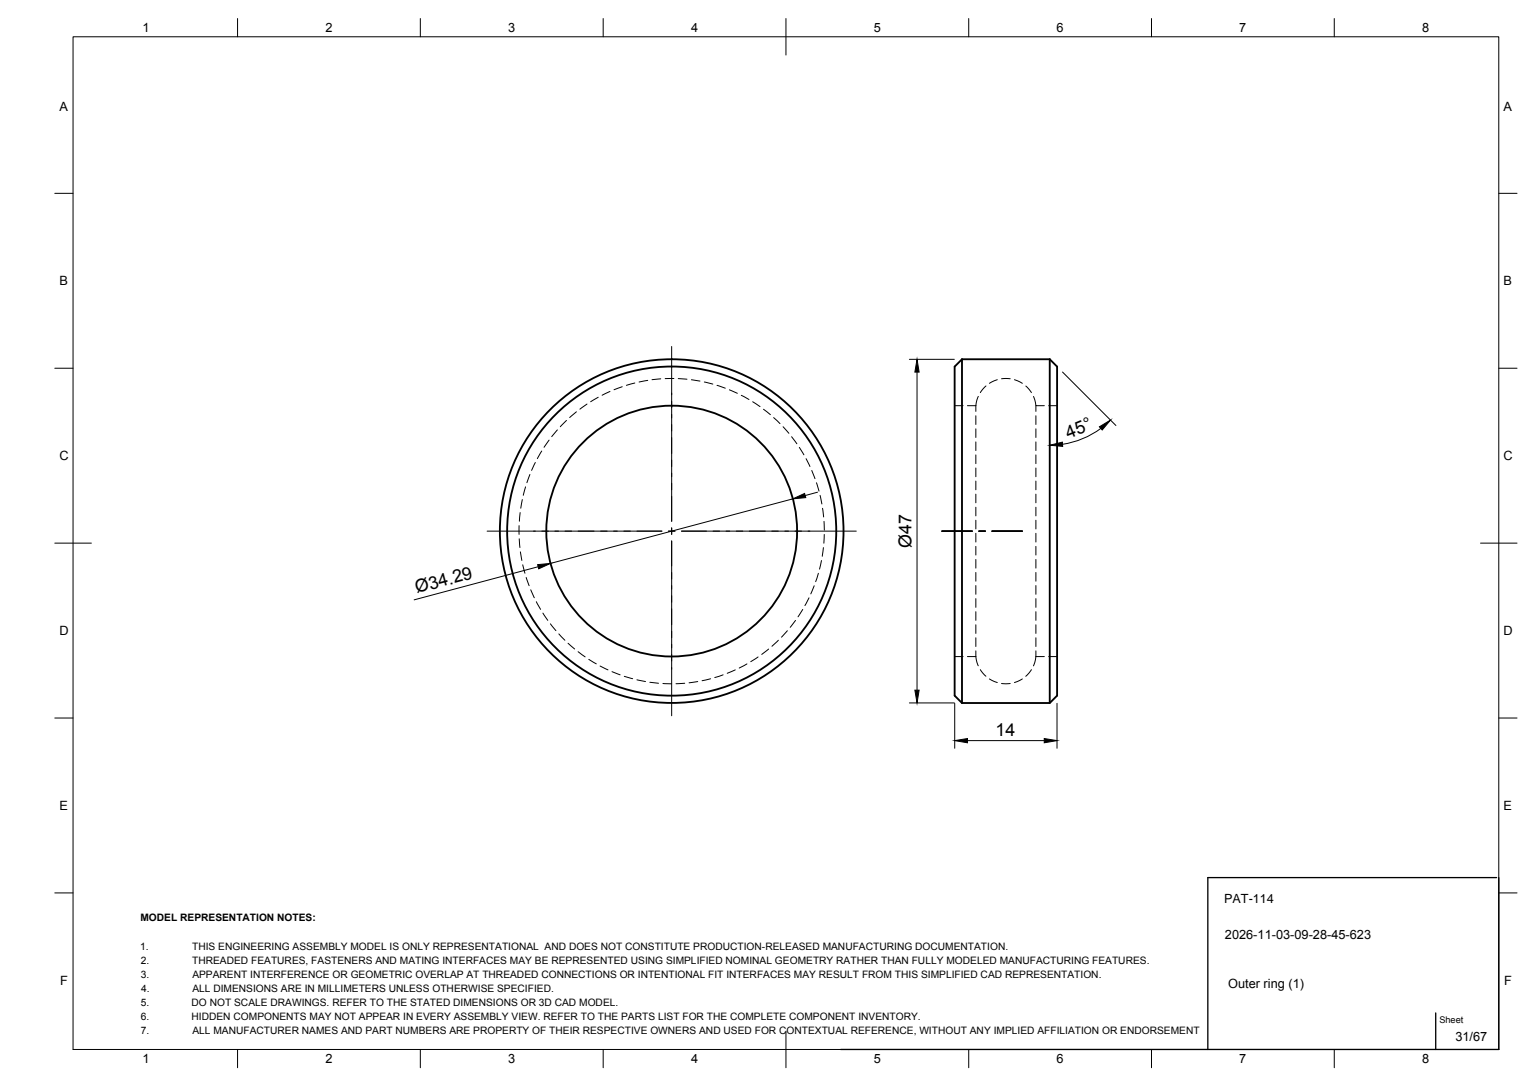
ISO-10303-21;
HEADER;
/* Generated by software containing ST-Developer
 * from STEP Tools, Inc. (www.steptools.com) 
 */

FILE_DESCRIPTION(
/* description */ ('Two-stage gear reducer in split housing'),
/* implementation_level */ '2;1');

FILE_NAME(
/* name */ 'Outer ring (1).step',
/* time_stamp */ '2026-10-28T03:22:31-07:00',
/* author */ (''),
/* organization */ (''),
/* preprocessor_version */ 'ST-DEVELOPER v20.2',
/* originating_system */ 'Autodesk Translation Framework v15.17.0.0',
/* authorisation */ '');

FILE_SCHEMA (('AUTOMOTIVE_DESIGN { 1 0 10303 214 3 1 1 }'));
ENDSEC;

DATA;
#10=MECHANICAL_DESIGN_GEOMETRIC_PRESENTATION_REPRESENTATION('',(#1264),#73366);
#1100=TOROIDAL_SURFACE('',#17566,1.675,0.412776);
#1110=CONICAL_SURFACE('',#17577,2.3,0.785398163397449);
#1111=CONICAL_SURFACE('',#17581,2.3,0.785398163397449);
#1145=SHAPE_REPRESENTATION_RELATIONSHIP('SRR','None',#73634,#1201);
#1201=ADVANCED_BREP_SHAPE_REPRESENTATION('',(#1334),#73330);
#1264=STYLED_ITEM('',(#73988),#1334);
#1334=MANIFOLD_SOLID_BREP('Body1',#16153);
#1530=FACE_BOUND('',#3428,.T.);
#1531=FACE_BOUND('',#3433,.T.);
#1773=PLANE('',#17574);
#1774=PLANE('',#17583);
#2356=FACE_OUTER_BOUND('',#3425,.T.);
#2357=FACE_OUTER_BOUND('',#3426,.T.);
#2358=FACE_OUTER_BOUND('',#3427,.T.);
#2359=FACE_OUTER_BOUND('',#3429,.T.);
#2360=FACE_OUTER_BOUND('',#3430,.T.);
#2361=FACE_OUTER_BOUND('',#3431,.T.);
#2362=FACE_OUTER_BOUND('',#3432,.T.);
#2363=FACE_OUTER_BOUND('',#3434,.T.);
#3425=EDGE_LOOP('',(#12045,#12046,#12047,#12048,#12049,#12050));
#3426=EDGE_LOOP('',(#12051,#12052,#12053,#12054,#12055));
#3427=EDGE_LOOP('',(#12056));
#3428=EDGE_LOOP('',(#12057));
#3429=EDGE_LOOP('',(#12058,#12059,#12060,#12061));
#3430=EDGE_LOOP('',(#12062,#12063,#12064,#12065));
#3431=EDGE_LOOP('',(#12066,#12067,#12068,#12069));
#3432=EDGE_LOOP('',(#12070));
#3433=EDGE_LOOP('',(#12071));
#3434=EDGE_LOOP('',(#12072,#12073,#12074,#12075,#12076));
#4444=LINE('',#24756,#5468);
#4445=LINE('',#24765,#5469);
#4446=LINE('',#24769,#5470);
#4447=LINE('',#24773,#5471);
#4448=LINE('',#24776,#5472);
#5468=VECTOR('',#20370,1.71469);
#5469=VECTOR('',#20381,2.3);
#5470=VECTOR('',#20386,2.35);
#5471=VECTOR('',#20391,2.3);
#5472=VECTOR('',#20396,1.71469);
#6471=CIRCLE('',#17567,1.71469);
#6472=CIRCLE('',#17568,1.71469);
#6473=CIRCLE('',#17569,0.412776);
#6474=CIRCLE('',#17570,1.71469);
#6475=CIRCLE('',#17571,1.71469);
#6476=CIRCLE('',#17573,1.71469);
#6477=CIRCLE('',#17575,2.25);
#6478=CIRCLE('',#17576,1.71469);
#6479=CIRCLE('',#17578,2.35);
#6480=CIRCLE('',#17580,2.35);
#6481=CIRCLE('',#17582,2.25);
#7343=VERTEX_POINT('',#24744);
#7344=VERTEX_POINT('',#24745);
#7345=VERTEX_POINT('',#24748);
#7346=VERTEX_POINT('',#24750);
#7347=VERTEX_POINT('',#24754);
#7348=VERTEX_POINT('',#24758);
#7349=VERTEX_POINT('',#24760);
#7350=VERTEX_POINT('',#24763);
#7351=VERTEX_POINT('',#24767);
#7352=VERTEX_POINT('',#24771);
#9076=EDGE_CURVE('',#7343,#7344,#6471,.T.);
#9077=EDGE_CURVE('',#7344,#7343,#6472,.T.);
#9078=EDGE_CURVE('',#7344,#7345,#6473,.T.);
#9079=EDGE_CURVE('',#7346,#7345,#6474,.T.);
#9080=EDGE_CURVE('',#7345,#7346,#6475,.T.);
#9081=EDGE_CURVE('',#7347,#7347,#6476,.T.);
#9082=EDGE_CURVE('',#7347,#7346,#4444,.T.);
#9083=EDGE_CURVE('',#7348,#7348,#6477,.T.);
#9084=EDGE_CURVE('',#7349,#7349,#6478,.T.);
#9085=EDGE_CURVE('',#7350,#7350,#6479,.T.);
#9086=EDGE_CURVE('',#7350,#7348,#4445,.T.);
#9087=EDGE_CURVE('',#7351,#7351,#6480,.T.);
#9088=EDGE_CURVE('',#7351,#7350,#4446,.T.);
#9089=EDGE_CURVE('',#7352,#7352,#6481,.T.);
#9090=EDGE_CURVE('',#7352,#7351,#4447,.T.);
#9091=EDGE_CURVE('',#7343,#7349,#4448,.T.);
#12045=ORIENTED_EDGE('',*,*,#9076,.F.);
#12046=ORIENTED_EDGE('',*,*,#9077,.F.);
#12047=ORIENTED_EDGE('',*,*,#9078,.T.);
#12048=ORIENTED_EDGE('',*,*,#9079,.F.);
#12049=ORIENTED_EDGE('',*,*,#9080,.F.);
#12050=ORIENTED_EDGE('',*,*,#9078,.F.);
#12051=ORIENTED_EDGE('',*,*,#9081,.T.);
#12052=ORIENTED_EDGE('',*,*,#9082,.T.);
#12053=ORIENTED_EDGE('',*,*,#9079,.T.);
#12054=ORIENTED_EDGE('',*,*,#9080,.T.);
#12055=ORIENTED_EDGE('',*,*,#9082,.F.);
#12056=ORIENTED_EDGE('',*,*,#9083,.F.);
#12057=ORIENTED_EDGE('',*,*,#9084,.T.);
#12058=ORIENTED_EDGE('',*,*,#9085,.F.);
#12059=ORIENTED_EDGE('',*,*,#9086,.T.);
#12060=ORIENTED_EDGE('',*,*,#9083,.T.);
#12061=ORIENTED_EDGE('',*,*,#9086,.F.);
#12062=ORIENTED_EDGE('',*,*,#9087,.F.);
#12063=ORIENTED_EDGE('',*,*,#9088,.T.);
#12064=ORIENTED_EDGE('',*,*,#9085,.T.);
#12065=ORIENTED_EDGE('',*,*,#9088,.F.);
#12066=ORIENTED_EDGE('',*,*,#9089,.F.);
#12067=ORIENTED_EDGE('',*,*,#9090,.T.);
#12068=ORIENTED_EDGE('',*,*,#9087,.T.);
#12069=ORIENTED_EDGE('',*,*,#9090,.F.);
#12070=ORIENTED_EDGE('',*,*,#9089,.T.);
#12071=ORIENTED_EDGE('',*,*,#9081,.F.);
#12072=ORIENTED_EDGE('',*,*,#9076,.T.);
#12073=ORIENTED_EDGE('',*,*,#9077,.T.);
#12074=ORIENTED_EDGE('',*,*,#9091,.T.);
#12075=ORIENTED_EDGE('',*,*,#9084,.F.);
#12076=ORIENTED_EDGE('',*,*,#9091,.F.);
#15064=CYLINDRICAL_SURFACE('',#17572,1.71469);
#15065=CYLINDRICAL_SURFACE('',#17579,2.35);
#15066=CYLINDRICAL_SURFACE('',#17584,1.71469);
#15563=ADVANCED_FACE('',(#2356),#1100,.F.);
#15564=ADVANCED_FACE('',(#2357),#15064,.F.);
#15565=ADVANCED_FACE('',(#2358,#1530),#1773,.T.);
#15566=ADVANCED_FACE('',(#2359),#1110,.T.);
#15567=ADVANCED_FACE('',(#2360),#15065,.T.);
#15568=ADVANCED_FACE('',(#2361),#1111,.T.);
#15569=ADVANCED_FACE('',(#2362,#1531),#1774,.T.);
#15570=ADVANCED_FACE('',(#2363),#15066,.F.);
#16153=CLOSED_SHELL('',(#15563,#15564,#15565,#15566,#15567,#15568,#15569,
#15570));
#17565=AXIS2_PLACEMENT_3D('',#24742,#20352,#20353);
#17566=AXIS2_PLACEMENT_3D('',#24743,#20354,#20355);
#17567=AXIS2_PLACEMENT_3D('',#24746,#20356,#20357);
#17568=AXIS2_PLACEMENT_3D('',#24747,#20358,#20359);
#17569=AXIS2_PLACEMENT_3D('',#24749,#20360,#20361);
#17570=AXIS2_PLACEMENT_3D('',#24751,#20362,#20363);
#17571=AXIS2_PLACEMENT_3D('',#24752,#20364,#20365);
#17572=AXIS2_PLACEMENT_3D('',#24753,#20366,#20367);
#17573=AXIS2_PLACEMENT_3D('',#24755,#20368,#20369);
#17574=AXIS2_PLACEMENT_3D('',#24757,#20371,#20372);
#17575=AXIS2_PLACEMENT_3D('',#24759,#20373,#20374);
#17576=AXIS2_PLACEMENT_3D('',#24761,#20375,#20376);
#17577=AXIS2_PLACEMENT_3D('',#24762,#20377,#20378);
#17578=AXIS2_PLACEMENT_3D('',#24764,#20379,#20380);
#17579=AXIS2_PLACEMENT_3D('',#24766,#20382,#20383);
#17580=AXIS2_PLACEMENT_3D('',#24768,#20384,#20385);
#17581=AXIS2_PLACEMENT_3D('',#24770,#20387,#20388);
#17582=AXIS2_PLACEMENT_3D('',#24772,#20389,#20390);
#17583=AXIS2_PLACEMENT_3D('',#24774,#20392,#20393);
#17584=AXIS2_PLACEMENT_3D('',#24775,#20394,#20395);
#20352=DIRECTION('axis',(0.,0.,1.));
#20353=DIRECTION('refdir',(1.,0.,0.));
#20354=DIRECTION('center_axis',(0.,-1.,0.));
#20355=DIRECTION('ref_axis',(0.,0.,-1.));
#20356=DIRECTION('center_axis',(0.,-1.,0.));
#20357=DIRECTION('ref_axis',(1.,0.,0.));
#20358=DIRECTION('center_axis',(0.,-1.,0.));
#20359=DIRECTION('ref_axis',(1.,0.,0.));
#20360=DIRECTION('center_axis',(1.,0.,1.22464679914735E-16));
#20361=DIRECTION('ref_axis',(-1.22464679914735E-16,0.,1.));
#20362=DIRECTION('center_axis',(0.,1.,0.));
#20363=DIRECTION('ref_axis',(1.,0.,0.));
#20364=DIRECTION('center_axis',(0.,1.,0.));
#20365=DIRECTION('ref_axis',(1.,0.,0.));
#20366=DIRECTION('center_axis',(0.,-1.,0.));
#20367=DIRECTION('ref_axis',(1.,0.,0.));
#20368=DIRECTION('center_axis',(0.,-1.,0.));
#20369=DIRECTION('ref_axis',(1.,0.,0.));
#20370=DIRECTION('',(0.,1.,0.));
#20371=DIRECTION('center_axis',(0.,1.,0.));
#20372=DIRECTION('ref_axis',(0.,0.,1.));
#20373=DIRECTION('center_axis',(0.,-1.,0.));
#20374=DIRECTION('ref_axis',(1.,0.,0.));
#20375=DIRECTION('center_axis',(0.,-1.,0.));
#20376=DIRECTION('ref_axis',(1.,0.,0.));
#20377=DIRECTION('center_axis',(0.,-1.,0.));
#20378=DIRECTION('ref_axis',(1.,0.,0.));
#20379=DIRECTION('center_axis',(0.,-1.,0.));
#20380=DIRECTION('ref_axis',(1.,0.,0.));
#20381=DIRECTION('',(0.707106781186548,0.707106781186547,8.65956056235494E-17));
#20382=DIRECTION('center_axis',(0.,-1.,0.));
#20383=DIRECTION('ref_axis',(1.,0.,0.));
#20384=DIRECTION('center_axis',(0.,-1.,0.));
#20385=DIRECTION('ref_axis',(1.,0.,0.));
#20386=DIRECTION('',(0.,1.,0.));
#20387=DIRECTION('center_axis',(0.,1.,0.));
#20388=DIRECTION('ref_axis',(1.,0.,0.));
#20389=DIRECTION('center_axis',(0.,-1.,0.));
#20390=DIRECTION('ref_axis',(1.,0.,0.));
#20391=DIRECTION('',(-0.707106781186548,0.707106781186547,-8.65956056235494E-17));
#20392=DIRECTION('center_axis',(0.,-1.,0.));
#20393=DIRECTION('ref_axis',(0.,0.,-1.));
#20394=DIRECTION('center_axis',(0.,-1.,0.));
#20395=DIRECTION('ref_axis',(1.,0.,0.));
#20396=DIRECTION('',(0.,1.,0.));
#24742=CARTESIAN_POINT('',(0.,0.,0.));
#24743=CARTESIAN_POINT('Origin',(0.,0.,0.));
#24744=CARTESIAN_POINT('',(-1.71469,0.410863395882378,-2.09988962002998E-16));
#24745=CARTESIAN_POINT('',(-2.09988962002998E-16,0.410863395882378,1.71469));
#24746=CARTESIAN_POINT('Origin',(0.,0.410863395882378,0.));
#24747=CARTESIAN_POINT('Origin',(0.,0.410863395882378,0.));
#24748=CARTESIAN_POINT('',(-2.09988962002998E-16,-0.410863395882378,1.71469));
#24749=CARTESIAN_POINT('Origin',(-2.05128338857182E-16,0.,1.675));
#24750=CARTESIAN_POINT('',(-1.71469,-0.410863395882378,2.09988962002998E-16));
#24751=CARTESIAN_POINT('Origin',(0.,-0.410863395882378,0.));
#24752=CARTESIAN_POINT('Origin',(0.,-0.410863395882378,0.));
#24753=CARTESIAN_POINT('Origin',(0.,0.,0.));
#24754=CARTESIAN_POINT('',(-1.71469,-0.7,-2.09988962002998E-16));
#24755=CARTESIAN_POINT('Origin',(0.,-0.7,0.));
#24756=CARTESIAN_POINT('',(-1.71469,0.,-2.09988962002998E-16));
#24757=CARTESIAN_POINT('Origin',(2.25,0.7,0.));
#24758=CARTESIAN_POINT('',(-2.25,0.7,-2.75545529808154E-16));
#24759=CARTESIAN_POINT('Origin',(0.,0.7,0.));
#24760=CARTESIAN_POINT('',(-1.71469,0.7,-2.09988962002998E-16));
#24761=CARTESIAN_POINT('Origin',(0.,0.7,0.));
#24762=CARTESIAN_POINT('Origin',(0.,0.65,0.));
#24763=CARTESIAN_POINT('',(-2.35,0.6,-2.87791997799628E-16));
#24764=CARTESIAN_POINT('Origin',(0.,0.6,0.));
#24765=CARTESIAN_POINT('',(-2.3,0.65,-2.81668763803891E-16));
#24766=CARTESIAN_POINT('Origin',(0.,0.,0.));
#24767=CARTESIAN_POINT('',(-2.35,-0.6,-2.87791997799628E-16));
#24768=CARTESIAN_POINT('Origin',(0.,-0.6,0.));
#24769=CARTESIAN_POINT('',(-2.35,0.,-2.87791997799628E-16));
#24770=CARTESIAN_POINT('Origin',(0.,-0.65,0.));
#24771=CARTESIAN_POINT('',(-2.25,-0.7,-2.75545529808154E-16));
#24772=CARTESIAN_POINT('Origin',(0.,-0.7,0.));
#24773=CARTESIAN_POINT('',(-2.3,-0.65,-2.81668763803891E-16));
#24774=CARTESIAN_POINT('Origin',(1.71469,-0.7,0.));
#24775=CARTESIAN_POINT('Origin',(0.,0.,0.));
#24776=CARTESIAN_POINT('',(-1.71469,0.,-2.09988962002998E-16));
#73266=UNCERTAINTY_MEASURE_WITH_UNIT(LENGTH_MEASURE(0.001),#73367,
'DISTANCE_ACCURACY_VALUE',
'Maximum model space distance between geometric entities at asserted c
onnectivities');
#73302=UNCERTAINTY_MEASURE_WITH_UNIT(LENGTH_MEASURE(0.001),#73367,
'DISTANCE_ACCURACY_VALUE',
'Maximum model space distance between geometric entities at asserted c
onnectivities');
#73330=(
GEOMETRIC_REPRESENTATION_CONTEXT(3)
GLOBAL_UNCERTAINTY_ASSIGNED_CONTEXT((#73266))
GLOBAL_UNIT_ASSIGNED_CONTEXT((#73367,#73369,#73370))
REPRESENTATION_CONTEXT('','3D')
);
#73366=(
GEOMETRIC_REPRESENTATION_CONTEXT(3)
GLOBAL_UNCERTAINTY_ASSIGNED_CONTEXT((#73302))
GLOBAL_UNIT_ASSIGNED_CONTEXT((#73367,#73369,#73370))
REPRESENTATION_CONTEXT('','3D')
);
#73367=(
LENGTH_UNIT()
NAMED_UNIT(*)
SI_UNIT(.CENTI.,.METRE.)
);
#73369=(
NAMED_UNIT(*)
PLANE_ANGLE_UNIT()
SI_UNIT($,.RADIAN.)
);
#73370=(
NAMED_UNIT(*)
SI_UNIT($,.STERADIAN.)
SOLID_ANGLE_UNIT()
);
#73398=SHAPE_DEFINITION_REPRESENTATION(#73466,#73634);
#73466=PRODUCT_DEFINITION_SHAPE('',$,#73698);
#73634=SHAPE_REPRESENTATION('',(#17565),#73330);
#73670=PRODUCT_DEFINITION_CONTEXT('part definition',#73861,'design');
#73698=PRODUCT_DEFINITION('Outer ring (1)','Outer ring (1)',#73761,#73670);
#73761=PRODUCT_DEFINITION_FORMATION('',$,#73890);
#73861=APPLICATION_CONTEXT(
'Core Data for Automotive Mechanical Design Process');
#73862=PRODUCT_CONTEXT('part definition',#73861,'mechanical');
#73890=PRODUCT('Outer ring (1)','Outer ring (1)','Outer ring (1)',(#73862));
#73982=COLOUR_RGB('Grey',0.48,0.52,0.57);
#73983=FILL_AREA_STYLE_COLOUR('',#73982);
#73984=FILL_AREA_STYLE('',(#73983));
#73985=SURFACE_STYLE_FILL_AREA(#73984);
#73986=SURFACE_SIDE_STYLE('',(#73985));
#73987=SURFACE_STYLE_USAGE(.BOTH.,#73986);
#73988=PRESENTATION_STYLE_ASSIGNMENT((#73987));
ENDSEC;
END-ISO-10303-21;
